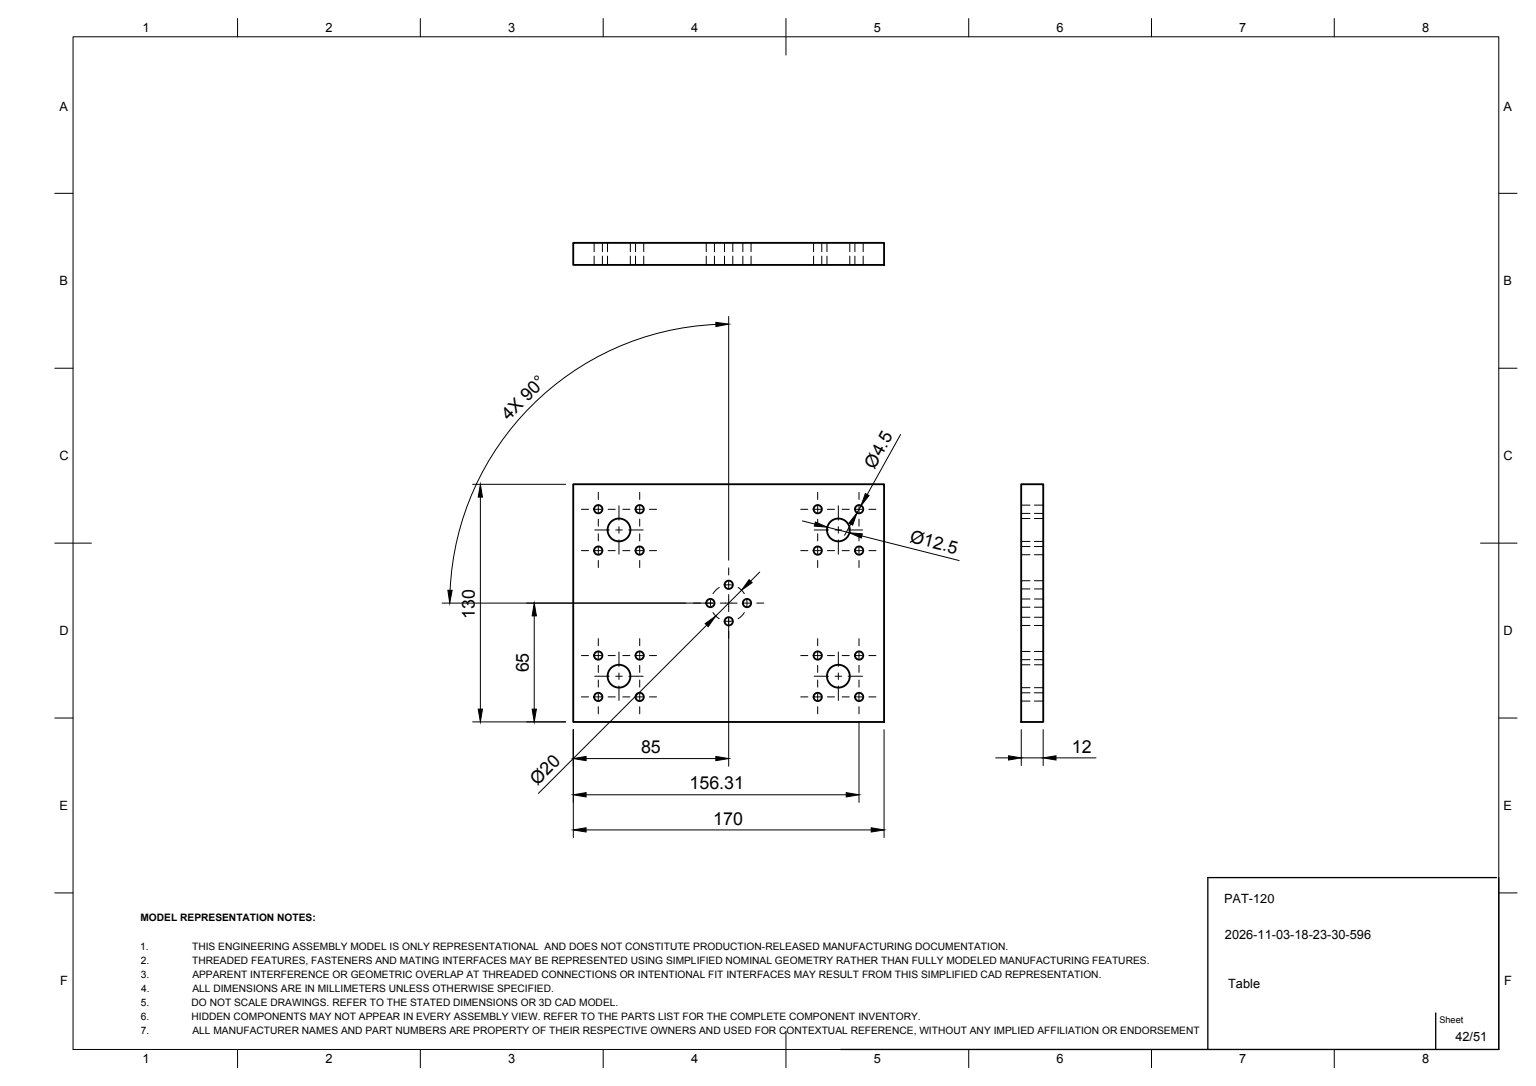
ISO-10303-21;
HEADER;
/* Generated by software containing ST-Developer
 * from STEP Tools, Inc. (www.steptools.com) 
 */

FILE_DESCRIPTION(
/* description */ ('Vibration shaker table dummy'),
/* implementation_level */ '2;1');

FILE_NAME(
/* name */ 'Table.step',
/* time_stamp */ '2026-10-27T10:55:14-07:00',
/* author */ (''),
/* organization */ (''),
/* preprocessor_version */ 'ST-DEVELOPER v20.2',
/* originating_system */ 'Autodesk Translation Framework v15.17.0.0',
/* authorisation */ '');

FILE_SCHEMA (('AUTOMOTIVE_DESIGN { 1 0 10303 214 3 1 1 }'));
ENDSEC;

DATA;
#10=MECHANICAL_DESIGN_GEOMETRIC_PRESENTATION_REPRESENTATION('',(#723),#22394);
#631=SHAPE_REPRESENTATION_RELATIONSHIP('SRR','None',#22678,#677);
#677=ADVANCED_BREP_SHAPE_REPRESENTATION('',(#767),#22384);
#723=STYLED_ITEM('',(#22975),#767);
#767=MANIFOLD_SOLID_BREP('Body1',#9243);
#959=FACE_BOUND('',#2405,.T.);
#960=FACE_BOUND('',#2406,.T.);
#961=FACE_BOUND('',#2407,.T.);
#962=FACE_BOUND('',#2408,.T.);
#963=FACE_BOUND('',#2409,.T.);
#964=FACE_BOUND('',#2410,.T.);
#965=FACE_BOUND('',#2411,.T.);
#966=FACE_BOUND('',#2412,.T.);
#967=FACE_BOUND('',#2413,.T.);
#968=FACE_BOUND('',#2414,.T.);
#969=FACE_BOUND('',#2415,.T.);
#970=FACE_BOUND('',#2416,.T.);
#971=FACE_BOUND('',#2417,.T.);
#972=FACE_BOUND('',#2418,.T.);
#973=FACE_BOUND('',#2419,.T.);
#974=FACE_BOUND('',#2420,.T.);
#975=FACE_BOUND('',#2421,.T.);
#976=FACE_BOUND('',#2422,.T.);
#977=FACE_BOUND('',#2423,.T.);
#978=FACE_BOUND('',#2424,.T.);
#979=FACE_BOUND('',#2425,.T.);
#980=FACE_BOUND('',#2426,.T.);
#981=FACE_BOUND('',#2427,.T.);
#982=FACE_BOUND('',#2428,.T.);
#983=FACE_BOUND('',#2430,.T.);
#984=FACE_BOUND('',#2431,.T.);
#985=FACE_BOUND('',#2432,.T.);
#986=FACE_BOUND('',#2433,.T.);
#987=FACE_BOUND('',#2434,.T.);
#988=FACE_BOUND('',#2435,.T.);
#989=FACE_BOUND('',#2436,.T.);
#990=FACE_BOUND('',#2437,.T.);
#991=FACE_BOUND('',#2438,.T.);
#992=FACE_BOUND('',#2439,.T.);
#993=FACE_BOUND('',#2440,.T.);
#994=FACE_BOUND('',#2441,.T.);
#995=FACE_BOUND('',#2442,.T.);
#996=FACE_BOUND('',#2443,.T.);
#997=FACE_BOUND('',#2444,.T.);
#998=FACE_BOUND('',#2445,.T.);
#999=FACE_BOUND('',#2446,.T.);
#1000=FACE_BOUND('',#2447,.T.);
#1001=FACE_BOUND('',#2448,.T.);
#1002=FACE_BOUND('',#2449,.T.);
#1003=FACE_BOUND('',#2450,.T.);
#1004=FACE_BOUND('',#2451,.T.);
#1005=FACE_BOUND('',#2452,.T.);
#1006=FACE_BOUND('',#2453,.T.);
#1272=PLANE('',#10511);
#1273=PLANE('',#10512);
#1274=PLANE('',#10513);
#1275=PLANE('',#10514);
#1276=PLANE('',#10515);
#1277=PLANE('',#10516);
#1694=FACE_OUTER_BOUND('',#2376,.T.);
#1695=FACE_OUTER_BOUND('',#2377,.T.);
#1696=FACE_OUTER_BOUND('',#2378,.T.);
#1697=FACE_OUTER_BOUND('',#2379,.T.);
#1698=FACE_OUTER_BOUND('',#2380,.T.);
#1699=FACE_OUTER_BOUND('',#2381,.T.);
#1700=FACE_OUTER_BOUND('',#2382,.T.);
#1701=FACE_OUTER_BOUND('',#2383,.T.);
#1702=FACE_OUTER_BOUND('',#2384,.T.);
#1703=FACE_OUTER_BOUND('',#2385,.T.);
#1704=FACE_OUTER_BOUND('',#2386,.T.);
#1705=FACE_OUTER_BOUND('',#2387,.T.);
#1706=FACE_OUTER_BOUND('',#2388,.T.);
#1707=FACE_OUTER_BOUND('',#2389,.T.);
#1708=FACE_OUTER_BOUND('',#2390,.T.);
#1709=FACE_OUTER_BOUND('',#2391,.T.);
#1710=FACE_OUTER_BOUND('',#2392,.T.);
#1711=FACE_OUTER_BOUND('',#2393,.T.);
#1712=FACE_OUTER_BOUND('',#2394,.T.);
#1713=FACE_OUTER_BOUND('',#2395,.T.);
#1714=FACE_OUTER_BOUND('',#2396,.T.);
#1715=FACE_OUTER_BOUND('',#2397,.T.);
#1716=FACE_OUTER_BOUND('',#2398,.T.);
#1717=FACE_OUTER_BOUND('',#2399,.T.);
#1718=FACE_OUTER_BOUND('',#2400,.T.);
#1719=FACE_OUTER_BOUND('',#2401,.T.);
#1720=FACE_OUTER_BOUND('',#2402,.T.);
#1721=FACE_OUTER_BOUND('',#2403,.T.);
#1722=FACE_OUTER_BOUND('',#2404,.T.);
#1723=FACE_OUTER_BOUND('',#2429,.T.);
#2376=EDGE_LOOP('',(#7758,#7759,#7760,#7761));
#2377=EDGE_LOOP('',(#7762,#7763,#7764,#7765));
#2378=EDGE_LOOP('',(#7766,#7767,#7768,#7769));
#2379=EDGE_LOOP('',(#7770,#7771,#7772,#7773));
#2380=EDGE_LOOP('',(#7774,#7775,#7776,#7777));
#2381=EDGE_LOOP('',(#7778,#7779,#7780,#7781));
#2382=EDGE_LOOP('',(#7782,#7783,#7784,#7785));
#2383=EDGE_LOOP('',(#7786,#7787,#7788,#7789));
#2384=EDGE_LOOP('',(#7790,#7791,#7792,#7793));
#2385=EDGE_LOOP('',(#7794,#7795,#7796,#7797));
#2386=EDGE_LOOP('',(#7798,#7799,#7800,#7801));
#2387=EDGE_LOOP('',(#7802,#7803,#7804,#7805));
#2388=EDGE_LOOP('',(#7806,#7807,#7808,#7809));
#2389=EDGE_LOOP('',(#7810,#7811,#7812,#7813));
#2390=EDGE_LOOP('',(#7814,#7815,#7816,#7817));
#2391=EDGE_LOOP('',(#7818,#7819,#7820,#7821));
#2392=EDGE_LOOP('',(#7822,#7823,#7824,#7825));
#2393=EDGE_LOOP('',(#7826,#7827,#7828,#7829));
#2394=EDGE_LOOP('',(#7830,#7831,#7832,#7833));
#2395=EDGE_LOOP('',(#7834,#7835,#7836,#7837));
#2396=EDGE_LOOP('',(#7838,#7839,#7840,#7841));
#2397=EDGE_LOOP('',(#7842,#7843,#7844,#7845));
#2398=EDGE_LOOP('',(#7846,#7847,#7848,#7849));
#2399=EDGE_LOOP('',(#7850,#7851,#7852,#7853));
#2400=EDGE_LOOP('',(#7854,#7855,#7856,#7857));
#2401=EDGE_LOOP('',(#7858,#7859,#7860,#7861));
#2402=EDGE_LOOP('',(#7862,#7863,#7864,#7865));
#2403=EDGE_LOOP('',(#7866,#7867,#7868,#7869));
#2404=EDGE_LOOP('',(#7870,#7871,#7872,#7873));
#2405=EDGE_LOOP('',(#7874));
#2406=EDGE_LOOP('',(#7875));
#2407=EDGE_LOOP('',(#7876));
#2408=EDGE_LOOP('',(#7877));
#2409=EDGE_LOOP('',(#7878));
#2410=EDGE_LOOP('',(#7879));
#2411=EDGE_LOOP('',(#7880));
#2412=EDGE_LOOP('',(#7881));
#2413=EDGE_LOOP('',(#7882));
#2414=EDGE_LOOP('',(#7883));
#2415=EDGE_LOOP('',(#7884));
#2416=EDGE_LOOP('',(#7885));
#2417=EDGE_LOOP('',(#7886));
#2418=EDGE_LOOP('',(#7887));
#2419=EDGE_LOOP('',(#7888));
#2420=EDGE_LOOP('',(#7889));
#2421=EDGE_LOOP('',(#7890));
#2422=EDGE_LOOP('',(#7891));
#2423=EDGE_LOOP('',(#7892));
#2424=EDGE_LOOP('',(#7893));
#2425=EDGE_LOOP('',(#7894));
#2426=EDGE_LOOP('',(#7895));
#2427=EDGE_LOOP('',(#7896));
#2428=EDGE_LOOP('',(#7897));
#2429=EDGE_LOOP('',(#7898,#7899,#7900,#7901));
#2430=EDGE_LOOP('',(#7902));
#2431=EDGE_LOOP('',(#7903));
#2432=EDGE_LOOP('',(#7904));
#2433=EDGE_LOOP('',(#7905));
#2434=EDGE_LOOP('',(#7906));
#2435=EDGE_LOOP('',(#7907));
#2436=EDGE_LOOP('',(#7908));
#2437=EDGE_LOOP('',(#7909));
#2438=EDGE_LOOP('',(#7910));
#2439=EDGE_LOOP('',(#7911));
#2440=EDGE_LOOP('',(#7912));
#2441=EDGE_LOOP('',(#7913));
#2442=EDGE_LOOP('',(#7914));
#2443=EDGE_LOOP('',(#7915));
#2444=EDGE_LOOP('',(#7916));
#2445=EDGE_LOOP('',(#7917));
#2446=EDGE_LOOP('',(#7918));
#2447=EDGE_LOOP('',(#7919));
#2448=EDGE_LOOP('',(#7920));
#2449=EDGE_LOOP('',(#7921));
#2450=EDGE_LOOP('',(#7922));
#2451=EDGE_LOOP('',(#7923));
#2452=EDGE_LOOP('',(#7924));
#2453=EDGE_LOOP('',(#7925));
#3085=LINE('',#21382,#3704);
#3086=LINE('',#21388,#3705);
#3087=LINE('',#21394,#3706);
#3088=LINE('',#21400,#3707);
#3089=LINE('',#21406,#3708);
#3090=LINE('',#21412,#3709);
#3091=LINE('',#21418,#3710);
#3092=LINE('',#21424,#3711);
#3093=LINE('',#21430,#3712);
#3094=LINE('',#21436,#3713);
#3095=LINE('',#21442,#3714);
#3096=LINE('',#21448,#3715);
#3097=LINE('',#21454,#3716);
#3098=LINE('',#21460,#3717);
#3099=LINE('',#21466,#3718);
#3100=LINE('',#21472,#3719);
#3101=LINE('',#21478,#3720);
#3102=LINE('',#21484,#3721);
#3103=LINE('',#21490,#3722);
#3104=LINE('',#21496,#3723);
#3105=LINE('',#21502,#3724);
#3106=LINE('',#21508,#3725);
#3107=LINE('',#21514,#3726);
#3108=LINE('',#21520,#3727);
#3109=LINE('',#21525,#3728);
#3110=LINE('',#21527,#3729);
#3111=LINE('',#21529,#3730);
#3112=LINE('',#21530,#3731);
#3113=LINE('',#21533,#3732);
#3114=LINE('',#21535,#3733);
#3115=LINE('',#21536,#3734);
#3116=LINE('',#21539,#3735);
#3117=LINE('',#21541,#3736);
#3118=LINE('',#21542,#3737);
#3119=LINE('',#21544,#3738);
#3120=LINE('',#21545,#3739);
#3704=VECTOR('',#12775,0.225);
#3705=VECTOR('',#12782,0.225);
#3706=VECTOR('',#12789,0.225);
#3707=VECTOR('',#12796,0.225);
#3708=VECTOR('',#12803,0.225);
#3709=VECTOR('',#12810,0.225);
#3710=VECTOR('',#12817,0.225);
#3711=VECTOR('',#12824,0.225);
#3712=VECTOR('',#12831,0.225);
#3713=VECTOR('',#12838,0.225);
#3714=VECTOR('',#12845,0.225);
#3715=VECTOR('',#12852,0.225);
#3716=VECTOR('',#12859,0.225);
#3717=VECTOR('',#12866,0.225);
#3718=VECTOR('',#12873,0.225);
#3719=VECTOR('',#12880,0.225);
#3720=VECTOR('',#12887,0.225);
#3721=VECTOR('',#12894,0.225);
#3722=VECTOR('',#12901,0.225);
#3723=VECTOR('',#12908,0.225);
#3724=VECTOR('',#12915,0.625);
#3725=VECTOR('',#12922,0.625);
#3726=VECTOR('',#12929,0.625);
#3727=VECTOR('',#12936,0.625);
#3728=VECTOR('',#12941,1.);
#3729=VECTOR('',#12942,1.);
#3730=VECTOR('',#12943,1.);
#3731=VECTOR('',#12944,1.);
#3732=VECTOR('',#12947,1.);
#3733=VECTOR('',#12948,1.);
#3734=VECTOR('',#12949,1.);
#3735=VECTOR('',#12952,1.);
#3736=VECTOR('',#12953,1.);
#3737=VECTOR('',#12954,1.);
#3738=VECTOR('',#12957,1.);
#3739=VECTOR('',#12958,1.);
#4149=CIRCLE('',#10440,0.225);
#4150=CIRCLE('',#10441,0.225);
#4151=CIRCLE('',#10443,0.225);
#4152=CIRCLE('',#10444,0.225);
#4153=CIRCLE('',#10446,0.225);
#4154=CIRCLE('',#10447,0.225);
#4155=CIRCLE('',#10449,0.225);
#4156=CIRCLE('',#10450,0.225);
#4157=CIRCLE('',#10452,0.225);
#4158=CIRCLE('',#10453,0.225);
#4159=CIRCLE('',#10455,0.225);
#4160=CIRCLE('',#10456,0.225);
#4161=CIRCLE('',#10458,0.225);
#4162=CIRCLE('',#10459,0.225);
#4163=CIRCLE('',#10461,0.225);
#4164=CIRCLE('',#10462,0.225);
#4165=CIRCLE('',#10464,0.225);
#4166=CIRCLE('',#10465,0.225);
#4167=CIRCLE('',#10467,0.225);
#4168=CIRCLE('',#10468,0.225);
#4169=CIRCLE('',#10470,0.225);
#4170=CIRCLE('',#10471,0.225);
#4171=CIRCLE('',#10473,0.225);
#4172=CIRCLE('',#10474,0.225);
#4173=CIRCLE('',#10476,0.225);
#4174=CIRCLE('',#10477,0.225);
#4175=CIRCLE('',#10479,0.225);
#4176=CIRCLE('',#10480,0.225);
#4177=CIRCLE('',#10482,0.225);
#4178=CIRCLE('',#10483,0.225);
#4179=CIRCLE('',#10485,0.225);
#4180=CIRCLE('',#10486,0.225);
#4181=CIRCLE('',#10488,0.225);
#4182=CIRCLE('',#10489,0.225);
#4183=CIRCLE('',#10491,0.225);
#4184=CIRCLE('',#10492,0.225);
#4185=CIRCLE('',#10494,0.225);
#4186=CIRCLE('',#10495,0.225);
#4187=CIRCLE('',#10497,0.225);
#4188=CIRCLE('',#10498,0.225);
#4189=CIRCLE('',#10500,0.625);
#4190=CIRCLE('',#10501,0.625);
#4191=CIRCLE('',#10503,0.625);
#4192=CIRCLE('',#10504,0.625);
#4193=CIRCLE('',#10506,0.625);
#4194=CIRCLE('',#10507,0.625);
#4195=CIRCLE('',#10509,0.625);
#4196=CIRCLE('',#10510,0.625);
#4868=VERTEX_POINT('',#21379);
#4869=VERTEX_POINT('',#21381);
#4870=VERTEX_POINT('',#21385);
#4871=VERTEX_POINT('',#21387);
#4872=VERTEX_POINT('',#21391);
#4873=VERTEX_POINT('',#21393);
#4874=VERTEX_POINT('',#21397);
#4875=VERTEX_POINT('',#21399);
#4876=VERTEX_POINT('',#21403);
#4877=VERTEX_POINT('',#21405);
#4878=VERTEX_POINT('',#21409);
#4879=VERTEX_POINT('',#21411);
#4880=VERTEX_POINT('',#21415);
#4881=VERTEX_POINT('',#21417);
#4882=VERTEX_POINT('',#21421);
#4883=VERTEX_POINT('',#21423);
#4884=VERTEX_POINT('',#21427);
#4885=VERTEX_POINT('',#21429);
#4886=VERTEX_POINT('',#21433);
#4887=VERTEX_POINT('',#21435);
#4888=VERTEX_POINT('',#21439);
#4889=VERTEX_POINT('',#21441);
#4890=VERTEX_POINT('',#21445);
#4891=VERTEX_POINT('',#21447);
#4892=VERTEX_POINT('',#21451);
#4893=VERTEX_POINT('',#21453);
#4894=VERTEX_POINT('',#21457);
#4895=VERTEX_POINT('',#21459);
#4896=VERTEX_POINT('',#21463);
#4897=VERTEX_POINT('',#21465);
#4898=VERTEX_POINT('',#21469);
#4899=VERTEX_POINT('',#21471);
#4900=VERTEX_POINT('',#21475);
#4901=VERTEX_POINT('',#21477);
#4902=VERTEX_POINT('',#21481);
#4903=VERTEX_POINT('',#21483);
#4904=VERTEX_POINT('',#21487);
#4905=VERTEX_POINT('',#21489);
#4906=VERTEX_POINT('',#21493);
#4907=VERTEX_POINT('',#21495);
#4908=VERTEX_POINT('',#21499);
#4909=VERTEX_POINT('',#21501);
#4910=VERTEX_POINT('',#21505);
#4911=VERTEX_POINT('',#21507);
#4912=VERTEX_POINT('',#21511);
#4913=VERTEX_POINT('',#21513);
#4914=VERTEX_POINT('',#21517);
#4915=VERTEX_POINT('',#21519);
#4916=VERTEX_POINT('',#21523);
#4917=VERTEX_POINT('',#21524);
#4918=VERTEX_POINT('',#21526);
#4919=VERTEX_POINT('',#21528);
#4920=VERTEX_POINT('',#21532);
#4921=VERTEX_POINT('',#21534);
#4922=VERTEX_POINT('',#21538);
#4923=VERTEX_POINT('',#21540);
#5872=EDGE_CURVE('',#4868,#4868,#4149,.T.);
#5873=EDGE_CURVE('',#4868,#4869,#3085,.T.);
#5874=EDGE_CURVE('',#4869,#4869,#4150,.T.);
#5875=EDGE_CURVE('',#4870,#4870,#4151,.T.);
#5876=EDGE_CURVE('',#4870,#4871,#3086,.T.);
#5877=EDGE_CURVE('',#4871,#4871,#4152,.T.);
#5878=EDGE_CURVE('',#4872,#4872,#4153,.T.);
#5879=EDGE_CURVE('',#4872,#4873,#3087,.T.);
#5880=EDGE_CURVE('',#4873,#4873,#4154,.T.);
#5881=EDGE_CURVE('',#4874,#4874,#4155,.T.);
#5882=EDGE_CURVE('',#4874,#4875,#3088,.T.);
#5883=EDGE_CURVE('',#4875,#4875,#4156,.T.);
#5884=EDGE_CURVE('',#4876,#4876,#4157,.T.);
#5885=EDGE_CURVE('',#4876,#4877,#3089,.T.);
#5886=EDGE_CURVE('',#4877,#4877,#4158,.T.);
#5887=EDGE_CURVE('',#4878,#4878,#4159,.T.);
#5888=EDGE_CURVE('',#4878,#4879,#3090,.T.);
#5889=EDGE_CURVE('',#4879,#4879,#4160,.T.);
#5890=EDGE_CURVE('',#4880,#4880,#4161,.T.);
#5891=EDGE_CURVE('',#4880,#4881,#3091,.T.);
#5892=EDGE_CURVE('',#4881,#4881,#4162,.T.);
#5893=EDGE_CURVE('',#4882,#4882,#4163,.T.);
#5894=EDGE_CURVE('',#4882,#4883,#3092,.T.);
#5895=EDGE_CURVE('',#4883,#4883,#4164,.T.);
#5896=EDGE_CURVE('',#4884,#4884,#4165,.T.);
#5897=EDGE_CURVE('',#4884,#4885,#3093,.T.);
#5898=EDGE_CURVE('',#4885,#4885,#4166,.T.);
#5899=EDGE_CURVE('',#4886,#4886,#4167,.T.);
#5900=EDGE_CURVE('',#4886,#4887,#3094,.T.);
#5901=EDGE_CURVE('',#4887,#4887,#4168,.T.);
#5902=EDGE_CURVE('',#4888,#4888,#4169,.T.);
#5903=EDGE_CURVE('',#4888,#4889,#3095,.T.);
#5904=EDGE_CURVE('',#4889,#4889,#4170,.T.);
#5905=EDGE_CURVE('',#4890,#4890,#4171,.T.);
#5906=EDGE_CURVE('',#4890,#4891,#3096,.T.);
#5907=EDGE_CURVE('',#4891,#4891,#4172,.T.);
#5908=EDGE_CURVE('',#4892,#4892,#4173,.T.);
#5909=EDGE_CURVE('',#4892,#4893,#3097,.T.);
#5910=EDGE_CURVE('',#4893,#4893,#4174,.T.);
#5911=EDGE_CURVE('',#4894,#4894,#4175,.T.);
#5912=EDGE_CURVE('',#4894,#4895,#3098,.T.);
#5913=EDGE_CURVE('',#4895,#4895,#4176,.T.);
#5914=EDGE_CURVE('',#4896,#4896,#4177,.T.);
#5915=EDGE_CURVE('',#4896,#4897,#3099,.T.);
#5916=EDGE_CURVE('',#4897,#4897,#4178,.T.);
#5917=EDGE_CURVE('',#4898,#4898,#4179,.T.);
#5918=EDGE_CURVE('',#4898,#4899,#3100,.T.);
#5919=EDGE_CURVE('',#4899,#4899,#4180,.T.);
#5920=EDGE_CURVE('',#4900,#4900,#4181,.T.);
#5921=EDGE_CURVE('',#4900,#4901,#3101,.T.);
#5922=EDGE_CURVE('',#4901,#4901,#4182,.T.);
#5923=EDGE_CURVE('',#4902,#4902,#4183,.T.);
#5924=EDGE_CURVE('',#4902,#4903,#3102,.T.);
#5925=EDGE_CURVE('',#4903,#4903,#4184,.T.);
#5926=EDGE_CURVE('',#4904,#4904,#4185,.T.);
#5927=EDGE_CURVE('',#4904,#4905,#3103,.T.);
#5928=EDGE_CURVE('',#4905,#4905,#4186,.T.);
#5929=EDGE_CURVE('',#4906,#4906,#4187,.T.);
#5930=EDGE_CURVE('',#4906,#4907,#3104,.T.);
#5931=EDGE_CURVE('',#4907,#4907,#4188,.T.);
#5932=EDGE_CURVE('',#4908,#4908,#4189,.T.);
#5933=EDGE_CURVE('',#4908,#4909,#3105,.T.);
#5934=EDGE_CURVE('',#4909,#4909,#4190,.T.);
#5935=EDGE_CURVE('',#4910,#4910,#4191,.T.);
#5936=EDGE_CURVE('',#4910,#4911,#3106,.T.);
#5937=EDGE_CURVE('',#4911,#4911,#4192,.T.);
#5938=EDGE_CURVE('',#4912,#4912,#4193,.T.);
#5939=EDGE_CURVE('',#4912,#4913,#3107,.T.);
#5940=EDGE_CURVE('',#4913,#4913,#4194,.T.);
#5941=EDGE_CURVE('',#4914,#4914,#4195,.T.);
#5942=EDGE_CURVE('',#4914,#4915,#3108,.T.);
#5943=EDGE_CURVE('',#4915,#4915,#4196,.T.);
#5944=EDGE_CURVE('',#4916,#4917,#3109,.T.);
#5945=EDGE_CURVE('',#4917,#4918,#3110,.T.);
#5946=EDGE_CURVE('',#4919,#4918,#3111,.T.);
#5947=EDGE_CURVE('',#4916,#4919,#3112,.T.);
#5948=EDGE_CURVE('',#4920,#4916,#3113,.T.);
#5949=EDGE_CURVE('',#4921,#4919,#3114,.T.);
#5950=EDGE_CURVE('',#4920,#4921,#3115,.T.);
#5951=EDGE_CURVE('',#4922,#4920,#3116,.T.);
#5952=EDGE_CURVE('',#4923,#4921,#3117,.T.);
#5953=EDGE_CURVE('',#4922,#4923,#3118,.T.);
#5954=EDGE_CURVE('',#4917,#4922,#3119,.T.);
#5955=EDGE_CURVE('',#4918,#4923,#3120,.T.);
#7758=ORIENTED_EDGE('',*,*,#5872,.F.);
#7759=ORIENTED_EDGE('',*,*,#5873,.T.);
#7760=ORIENTED_EDGE('',*,*,#5874,.F.);
#7761=ORIENTED_EDGE('',*,*,#5873,.F.);
#7762=ORIENTED_EDGE('',*,*,#5875,.F.);
#7763=ORIENTED_EDGE('',*,*,#5876,.T.);
#7764=ORIENTED_EDGE('',*,*,#5877,.F.);
#7765=ORIENTED_EDGE('',*,*,#5876,.F.);
#7766=ORIENTED_EDGE('',*,*,#5878,.F.);
#7767=ORIENTED_EDGE('',*,*,#5879,.T.);
#7768=ORIENTED_EDGE('',*,*,#5880,.F.);
#7769=ORIENTED_EDGE('',*,*,#5879,.F.);
#7770=ORIENTED_EDGE('',*,*,#5881,.F.);
#7771=ORIENTED_EDGE('',*,*,#5882,.T.);
#7772=ORIENTED_EDGE('',*,*,#5883,.F.);
#7773=ORIENTED_EDGE('',*,*,#5882,.F.);
#7774=ORIENTED_EDGE('',*,*,#5884,.F.);
#7775=ORIENTED_EDGE('',*,*,#5885,.T.);
#7776=ORIENTED_EDGE('',*,*,#5886,.F.);
#7777=ORIENTED_EDGE('',*,*,#5885,.F.);
#7778=ORIENTED_EDGE('',*,*,#5887,.F.);
#7779=ORIENTED_EDGE('',*,*,#5888,.T.);
#7780=ORIENTED_EDGE('',*,*,#5889,.F.);
#7781=ORIENTED_EDGE('',*,*,#5888,.F.);
#7782=ORIENTED_EDGE('',*,*,#5890,.F.);
#7783=ORIENTED_EDGE('',*,*,#5891,.T.);
#7784=ORIENTED_EDGE('',*,*,#5892,.F.);
#7785=ORIENTED_EDGE('',*,*,#5891,.F.);
#7786=ORIENTED_EDGE('',*,*,#5893,.F.);
#7787=ORIENTED_EDGE('',*,*,#5894,.T.);
#7788=ORIENTED_EDGE('',*,*,#5895,.F.);
#7789=ORIENTED_EDGE('',*,*,#5894,.F.);
#7790=ORIENTED_EDGE('',*,*,#5896,.F.);
#7791=ORIENTED_EDGE('',*,*,#5897,.T.);
#7792=ORIENTED_EDGE('',*,*,#5898,.F.);
#7793=ORIENTED_EDGE('',*,*,#5897,.F.);
#7794=ORIENTED_EDGE('',*,*,#5899,.F.);
#7795=ORIENTED_EDGE('',*,*,#5900,.T.);
#7796=ORIENTED_EDGE('',*,*,#5901,.F.);
#7797=ORIENTED_EDGE('',*,*,#5900,.F.);
#7798=ORIENTED_EDGE('',*,*,#5902,.F.);
#7799=ORIENTED_EDGE('',*,*,#5903,.T.);
#7800=ORIENTED_EDGE('',*,*,#5904,.F.);
#7801=ORIENTED_EDGE('',*,*,#5903,.F.);
#7802=ORIENTED_EDGE('',*,*,#5905,.F.);
#7803=ORIENTED_EDGE('',*,*,#5906,.T.);
#7804=ORIENTED_EDGE('',*,*,#5907,.F.);
#7805=ORIENTED_EDGE('',*,*,#5906,.F.);
#7806=ORIENTED_EDGE('',*,*,#5908,.F.);
#7807=ORIENTED_EDGE('',*,*,#5909,.T.);
#7808=ORIENTED_EDGE('',*,*,#5910,.F.);
#7809=ORIENTED_EDGE('',*,*,#5909,.F.);
#7810=ORIENTED_EDGE('',*,*,#5911,.F.);
#7811=ORIENTED_EDGE('',*,*,#5912,.T.);
#7812=ORIENTED_EDGE('',*,*,#5913,.F.);
#7813=ORIENTED_EDGE('',*,*,#5912,.F.);
#7814=ORIENTED_EDGE('',*,*,#5914,.F.);
#7815=ORIENTED_EDGE('',*,*,#5915,.T.);
#7816=ORIENTED_EDGE('',*,*,#5916,.F.);
#7817=ORIENTED_EDGE('',*,*,#5915,.F.);
#7818=ORIENTED_EDGE('',*,*,#5917,.F.);
#7819=ORIENTED_EDGE('',*,*,#5918,.T.);
#7820=ORIENTED_EDGE('',*,*,#5919,.F.);
#7821=ORIENTED_EDGE('',*,*,#5918,.F.);
#7822=ORIENTED_EDGE('',*,*,#5920,.F.);
#7823=ORIENTED_EDGE('',*,*,#5921,.T.);
#7824=ORIENTED_EDGE('',*,*,#5922,.F.);
#7825=ORIENTED_EDGE('',*,*,#5921,.F.);
#7826=ORIENTED_EDGE('',*,*,#5923,.F.);
#7827=ORIENTED_EDGE('',*,*,#5924,.T.);
#7828=ORIENTED_EDGE('',*,*,#5925,.F.);
#7829=ORIENTED_EDGE('',*,*,#5924,.F.);
#7830=ORIENTED_EDGE('',*,*,#5926,.F.);
#7831=ORIENTED_EDGE('',*,*,#5927,.T.);
#7832=ORIENTED_EDGE('',*,*,#5928,.F.);
#7833=ORIENTED_EDGE('',*,*,#5927,.F.);
#7834=ORIENTED_EDGE('',*,*,#5929,.F.);
#7835=ORIENTED_EDGE('',*,*,#5930,.T.);
#7836=ORIENTED_EDGE('',*,*,#5931,.F.);
#7837=ORIENTED_EDGE('',*,*,#5930,.F.);
#7838=ORIENTED_EDGE('',*,*,#5932,.F.);
#7839=ORIENTED_EDGE('',*,*,#5933,.T.);
#7840=ORIENTED_EDGE('',*,*,#5934,.F.);
#7841=ORIENTED_EDGE('',*,*,#5933,.F.);
#7842=ORIENTED_EDGE('',*,*,#5935,.F.);
#7843=ORIENTED_EDGE('',*,*,#5936,.T.);
#7844=ORIENTED_EDGE('',*,*,#5937,.F.);
#7845=ORIENTED_EDGE('',*,*,#5936,.F.);
#7846=ORIENTED_EDGE('',*,*,#5938,.F.);
#7847=ORIENTED_EDGE('',*,*,#5939,.T.);
#7848=ORIENTED_EDGE('',*,*,#5940,.F.);
#7849=ORIENTED_EDGE('',*,*,#5939,.F.);
#7850=ORIENTED_EDGE('',*,*,#5941,.F.);
#7851=ORIENTED_EDGE('',*,*,#5942,.T.);
#7852=ORIENTED_EDGE('',*,*,#5943,.F.);
#7853=ORIENTED_EDGE('',*,*,#5942,.F.);
#7854=ORIENTED_EDGE('',*,*,#5944,.T.);
#7855=ORIENTED_EDGE('',*,*,#5945,.T.);
#7856=ORIENTED_EDGE('',*,*,#5946,.F.);
#7857=ORIENTED_EDGE('',*,*,#5947,.F.);
#7858=ORIENTED_EDGE('',*,*,#5948,.T.);
#7859=ORIENTED_EDGE('',*,*,#5947,.T.);
#7860=ORIENTED_EDGE('',*,*,#5949,.F.);
#7861=ORIENTED_EDGE('',*,*,#5950,.F.);
#7862=ORIENTED_EDGE('',*,*,#5951,.T.);
#7863=ORIENTED_EDGE('',*,*,#5950,.T.);
#7864=ORIENTED_EDGE('',*,*,#5952,.F.);
#7865=ORIENTED_EDGE('',*,*,#5953,.F.);
#7866=ORIENTED_EDGE('',*,*,#5954,.T.);
#7867=ORIENTED_EDGE('',*,*,#5953,.T.);
#7868=ORIENTED_EDGE('',*,*,#5955,.F.);
#7869=ORIENTED_EDGE('',*,*,#5945,.F.);
#7870=ORIENTED_EDGE('',*,*,#5955,.T.);
#7871=ORIENTED_EDGE('',*,*,#5952,.T.);
#7872=ORIENTED_EDGE('',*,*,#5949,.T.);
#7873=ORIENTED_EDGE('',*,*,#5946,.T.);
#7874=ORIENTED_EDGE('',*,*,#5886,.T.);
#7875=ORIENTED_EDGE('',*,*,#5889,.T.);
#7876=ORIENTED_EDGE('',*,*,#5892,.T.);
#7877=ORIENTED_EDGE('',*,*,#5895,.T.);
#7878=ORIENTED_EDGE('',*,*,#5910,.T.);
#7879=ORIENTED_EDGE('',*,*,#5913,.T.);
#7880=ORIENTED_EDGE('',*,*,#5916,.T.);
#7881=ORIENTED_EDGE('',*,*,#5919,.T.);
#7882=ORIENTED_EDGE('',*,*,#5943,.T.);
#7883=ORIENTED_EDGE('',*,*,#5940,.T.);
#7884=ORIENTED_EDGE('',*,*,#5937,.T.);
#7885=ORIENTED_EDGE('',*,*,#5934,.T.);
#7886=ORIENTED_EDGE('',*,*,#5931,.T.);
#7887=ORIENTED_EDGE('',*,*,#5928,.T.);
#7888=ORIENTED_EDGE('',*,*,#5925,.T.);
#7889=ORIENTED_EDGE('',*,*,#5922,.T.);
#7890=ORIENTED_EDGE('',*,*,#5907,.T.);
#7891=ORIENTED_EDGE('',*,*,#5904,.T.);
#7892=ORIENTED_EDGE('',*,*,#5901,.T.);
#7893=ORIENTED_EDGE('',*,*,#5898,.T.);
#7894=ORIENTED_EDGE('',*,*,#5883,.T.);
#7895=ORIENTED_EDGE('',*,*,#5880,.T.);
#7896=ORIENTED_EDGE('',*,*,#5877,.T.);
#7897=ORIENTED_EDGE('',*,*,#5874,.T.);
#7898=ORIENTED_EDGE('',*,*,#5954,.F.);
#7899=ORIENTED_EDGE('',*,*,#5944,.F.);
#7900=ORIENTED_EDGE('',*,*,#5948,.F.);
#7901=ORIENTED_EDGE('',*,*,#5951,.F.);
#7902=ORIENTED_EDGE('',*,*,#5884,.T.);
#7903=ORIENTED_EDGE('',*,*,#5887,.T.);
#7904=ORIENTED_EDGE('',*,*,#5890,.T.);
#7905=ORIENTED_EDGE('',*,*,#5893,.T.);
#7906=ORIENTED_EDGE('',*,*,#5908,.T.);
#7907=ORIENTED_EDGE('',*,*,#5911,.T.);
#7908=ORIENTED_EDGE('',*,*,#5914,.T.);
#7909=ORIENTED_EDGE('',*,*,#5917,.T.);
#7910=ORIENTED_EDGE('',*,*,#5941,.T.);
#7911=ORIENTED_EDGE('',*,*,#5938,.T.);
#7912=ORIENTED_EDGE('',*,*,#5935,.T.);
#7913=ORIENTED_EDGE('',*,*,#5932,.T.);
#7914=ORIENTED_EDGE('',*,*,#5929,.T.);
#7915=ORIENTED_EDGE('',*,*,#5926,.T.);
#7916=ORIENTED_EDGE('',*,*,#5923,.T.);
#7917=ORIENTED_EDGE('',*,*,#5920,.T.);
#7918=ORIENTED_EDGE('',*,*,#5905,.T.);
#7919=ORIENTED_EDGE('',*,*,#5902,.T.);
#7920=ORIENTED_EDGE('',*,*,#5899,.T.);
#7921=ORIENTED_EDGE('',*,*,#5896,.T.);
#7922=ORIENTED_EDGE('',*,*,#5881,.T.);
#7923=ORIENTED_EDGE('',*,*,#5878,.T.);
#7924=ORIENTED_EDGE('',*,*,#5875,.T.);
#7925=ORIENTED_EDGE('',*,*,#5872,.T.);
#8634=CYLINDRICAL_SURFACE('',#10439,0.225);
#8635=CYLINDRICAL_SURFACE('',#10442,0.225);
#8636=CYLINDRICAL_SURFACE('',#10445,0.225);
#8637=CYLINDRICAL_SURFACE('',#10448,0.225);
#8638=CYLINDRICAL_SURFACE('',#10451,0.225);
#8639=CYLINDRICAL_SURFACE('',#10454,0.225);
#8640=CYLINDRICAL_SURFACE('',#10457,0.225);
#8641=CYLINDRICAL_SURFACE('',#10460,0.225);
#8642=CYLINDRICAL_SURFACE('',#10463,0.225);
#8643=CYLINDRICAL_SURFACE('',#10466,0.225);
#8644=CYLINDRICAL_SURFACE('',#10469,0.225);
#8645=CYLINDRICAL_SURFACE('',#10472,0.225);
#8646=CYLINDRICAL_SURFACE('',#10475,0.225);
#8647=CYLINDRICAL_SURFACE('',#10478,0.225);
#8648=CYLINDRICAL_SURFACE('',#10481,0.225);
#8649=CYLINDRICAL_SURFACE('',#10484,0.225);
#8650=CYLINDRICAL_SURFACE('',#10487,0.225);
#8651=CYLINDRICAL_SURFACE('',#10490,0.225);
#8652=CYLINDRICAL_SURFACE('',#10493,0.225);
#8653=CYLINDRICAL_SURFACE('',#10496,0.225);
#8654=CYLINDRICAL_SURFACE('',#10499,0.625);
#8655=CYLINDRICAL_SURFACE('',#10502,0.625);
#8656=CYLINDRICAL_SURFACE('',#10505,0.625);
#8657=CYLINDRICAL_SURFACE('',#10508,0.625);
#9059=ADVANCED_FACE('',(#1694),#8634,.F.);
#9060=ADVANCED_FACE('',(#1695),#8635,.F.);
#9061=ADVANCED_FACE('',(#1696),#8636,.F.);
#9062=ADVANCED_FACE('',(#1697),#8637,.F.);
#9063=ADVANCED_FACE('',(#1698),#8638,.F.);
#9064=ADVANCED_FACE('',(#1699),#8639,.F.);
#9065=ADVANCED_FACE('',(#1700),#8640,.F.);
#9066=ADVANCED_FACE('',(#1701),#8641,.F.);
#9067=ADVANCED_FACE('',(#1702),#8642,.F.);
#9068=ADVANCED_FACE('',(#1703),#8643,.F.);
#9069=ADVANCED_FACE('',(#1704),#8644,.F.);
#9070=ADVANCED_FACE('',(#1705),#8645,.F.);
#9071=ADVANCED_FACE('',(#1706),#8646,.F.);
#9072=ADVANCED_FACE('',(#1707),#8647,.F.);
#9073=ADVANCED_FACE('',(#1708),#8648,.F.);
#9074=ADVANCED_FACE('',(#1709),#8649,.F.);
#9075=ADVANCED_FACE('',(#1710),#8650,.F.);
#9076=ADVANCED_FACE('',(#1711),#8651,.F.);
#9077=ADVANCED_FACE('',(#1712),#8652,.F.);
#9078=ADVANCED_FACE('',(#1713),#8653,.F.);
#9079=ADVANCED_FACE('',(#1714),#8654,.F.);
#9080=ADVANCED_FACE('',(#1715),#8655,.F.);
#9081=ADVANCED_FACE('',(#1716),#8656,.F.);
#9082=ADVANCED_FACE('',(#1717),#8657,.F.);
#9083=ADVANCED_FACE('',(#1718),#1272,.T.);
#9084=ADVANCED_FACE('',(#1719),#1273,.T.);
#9085=ADVANCED_FACE('',(#1720),#1274,.T.);
#9086=ADVANCED_FACE('',(#1721),#1275,.T.);
#9087=ADVANCED_FACE('',(#1722,#959,#960,#961,#962,#963,#964,#965,#966,#967,
#968,#969,#970,#971,#972,#973,#974,#975,#976,#977,#978,#979,#980,#981,#982),
#1276,.T.);
#9088=ADVANCED_FACE('',(#1723,#983,#984,#985,#986,#987,#988,#989,#990,#991,
#992,#993,#994,#995,#996,#997,#998,#999,#1000,#1001,#1002,#1003,#1004,#1005,
#1006),#1277,.F.);
#9243=CLOSED_SHELL('',(#9059,#9060,#9061,#9062,#9063,#9064,#9065,#9066,
#9067,#9068,#9069,#9070,#9071,#9072,#9073,#9074,#9075,#9076,#9077,#9078,
#9079,#9080,#9081,#9082,#9083,#9084,#9085,#9086,#9087,#9088));
#10438=AXIS2_PLACEMENT_3D('',#21377,#12769,#12770);
#10439=AXIS2_PLACEMENT_3D('',#21378,#12771,#12772);
#10440=AXIS2_PLACEMENT_3D('',#21380,#12773,#12774);
#10441=AXIS2_PLACEMENT_3D('',#21383,#12776,#12777);
#10442=AXIS2_PLACEMENT_3D('',#21384,#12778,#12779);
#10443=AXIS2_PLACEMENT_3D('',#21386,#12780,#12781);
#10444=AXIS2_PLACEMENT_3D('',#21389,#12783,#12784);
#10445=AXIS2_PLACEMENT_3D('',#21390,#12785,#12786);
#10446=AXIS2_PLACEMENT_3D('',#21392,#12787,#12788);
#10447=AXIS2_PLACEMENT_3D('',#21395,#12790,#12791);
#10448=AXIS2_PLACEMENT_3D('',#21396,#12792,#12793);
#10449=AXIS2_PLACEMENT_3D('',#21398,#12794,#12795);
#10450=AXIS2_PLACEMENT_3D('',#21401,#12797,#12798);
#10451=AXIS2_PLACEMENT_3D('',#21402,#12799,#12800);
#10452=AXIS2_PLACEMENT_3D('',#21404,#12801,#12802);
#10453=AXIS2_PLACEMENT_3D('',#21407,#12804,#12805);
#10454=AXIS2_PLACEMENT_3D('',#21408,#12806,#12807);
#10455=AXIS2_PLACEMENT_3D('',#21410,#12808,#12809);
#10456=AXIS2_PLACEMENT_3D('',#21413,#12811,#12812);
#10457=AXIS2_PLACEMENT_3D('',#21414,#12813,#12814);
#10458=AXIS2_PLACEMENT_3D('',#21416,#12815,#12816);
#10459=AXIS2_PLACEMENT_3D('',#21419,#12818,#12819);
#10460=AXIS2_PLACEMENT_3D('',#21420,#12820,#12821);
#10461=AXIS2_PLACEMENT_3D('',#21422,#12822,#12823);
#10462=AXIS2_PLACEMENT_3D('',#21425,#12825,#12826);
#10463=AXIS2_PLACEMENT_3D('',#21426,#12827,#12828);
#10464=AXIS2_PLACEMENT_3D('',#21428,#12829,#12830);
#10465=AXIS2_PLACEMENT_3D('',#21431,#12832,#12833);
#10466=AXIS2_PLACEMENT_3D('',#21432,#12834,#12835);
#10467=AXIS2_PLACEMENT_3D('',#21434,#12836,#12837);
#10468=AXIS2_PLACEMENT_3D('',#21437,#12839,#12840);
#10469=AXIS2_PLACEMENT_3D('',#21438,#12841,#12842);
#10470=AXIS2_PLACEMENT_3D('',#21440,#12843,#12844);
#10471=AXIS2_PLACEMENT_3D('',#21443,#12846,#12847);
#10472=AXIS2_PLACEMENT_3D('',#21444,#12848,#12849);
#10473=AXIS2_PLACEMENT_3D('',#21446,#12850,#12851);
#10474=AXIS2_PLACEMENT_3D('',#21449,#12853,#12854);
#10475=AXIS2_PLACEMENT_3D('',#21450,#12855,#12856);
#10476=AXIS2_PLACEMENT_3D('',#21452,#12857,#12858);
#10477=AXIS2_PLACEMENT_3D('',#21455,#12860,#12861);
#10478=AXIS2_PLACEMENT_3D('',#21456,#12862,#12863);
#10479=AXIS2_PLACEMENT_3D('',#21458,#12864,#12865);
#10480=AXIS2_PLACEMENT_3D('',#21461,#12867,#12868);
#10481=AXIS2_PLACEMENT_3D('',#21462,#12869,#12870);
#10482=AXIS2_PLACEMENT_3D('',#21464,#12871,#12872);
#10483=AXIS2_PLACEMENT_3D('',#21467,#12874,#12875);
#10484=AXIS2_PLACEMENT_3D('',#21468,#12876,#12877);
#10485=AXIS2_PLACEMENT_3D('',#21470,#12878,#12879);
#10486=AXIS2_PLACEMENT_3D('',#21473,#12881,#12882);
#10487=AXIS2_PLACEMENT_3D('',#21474,#12883,#12884);
#10488=AXIS2_PLACEMENT_3D('',#21476,#12885,#12886);
#10489=AXIS2_PLACEMENT_3D('',#21479,#12888,#12889);
#10490=AXIS2_PLACEMENT_3D('',#21480,#12890,#12891);
#10491=AXIS2_PLACEMENT_3D('',#21482,#12892,#12893);
#10492=AXIS2_PLACEMENT_3D('',#21485,#12895,#12896);
#10493=AXIS2_PLACEMENT_3D('',#21486,#12897,#12898);
#10494=AXIS2_PLACEMENT_3D('',#21488,#12899,#12900);
#10495=AXIS2_PLACEMENT_3D('',#21491,#12902,#12903);
#10496=AXIS2_PLACEMENT_3D('',#21492,#12904,#12905);
#10497=AXIS2_PLACEMENT_3D('',#21494,#12906,#12907);
#10498=AXIS2_PLACEMENT_3D('',#21497,#12909,#12910);
#10499=AXIS2_PLACEMENT_3D('',#21498,#12911,#12912);
#10500=AXIS2_PLACEMENT_3D('',#21500,#12913,#12914);
#10501=AXIS2_PLACEMENT_3D('',#21503,#12916,#12917);
#10502=AXIS2_PLACEMENT_3D('',#21504,#12918,#12919);
#10503=AXIS2_PLACEMENT_3D('',#21506,#12920,#12921);
#10504=AXIS2_PLACEMENT_3D('',#21509,#12923,#12924);
#10505=AXIS2_PLACEMENT_3D('',#21510,#12925,#12926);
#10506=AXIS2_PLACEMENT_3D('',#21512,#12927,#12928);
#10507=AXIS2_PLACEMENT_3D('',#21515,#12930,#12931);
#10508=AXIS2_PLACEMENT_3D('',#21516,#12932,#12933);
#10509=AXIS2_PLACEMENT_3D('',#21518,#12934,#12935);
#10510=AXIS2_PLACEMENT_3D('',#21521,#12937,#12938);
#10511=AXIS2_PLACEMENT_3D('',#21522,#12939,#12940);
#10512=AXIS2_PLACEMENT_3D('',#21531,#12945,#12946);
#10513=AXIS2_PLACEMENT_3D('',#21537,#12950,#12951);
#10514=AXIS2_PLACEMENT_3D('',#21543,#12955,#12956);
#10515=AXIS2_PLACEMENT_3D('',#21546,#12959,#12960);
#10516=AXIS2_PLACEMENT_3D('',#21547,#12961,#12962);
#12769=DIRECTION('axis',(0.,0.,1.));
#12770=DIRECTION('refdir',(1.,0.,0.));
#12771=DIRECTION('center_axis',(0.,0.,1.));
#12772=DIRECTION('ref_axis',(1.,0.,0.));
#12773=DIRECTION('center_axis',(0.,0.,1.));
#12774=DIRECTION('ref_axis',(1.,0.,0.));
#12775=DIRECTION('',(0.,0.,1.));
#12776=DIRECTION('center_axis',(0.,0.,-1.));
#12777=DIRECTION('ref_axis',(1.,0.,0.));
#12778=DIRECTION('center_axis',(0.,0.,1.));
#12779=DIRECTION('ref_axis',(1.,0.,0.));
#12780=DIRECTION('center_axis',(0.,0.,1.));
#12781=DIRECTION('ref_axis',(1.,0.,0.));
#12782=DIRECTION('',(0.,0.,1.));
#12783=DIRECTION('center_axis',(0.,0.,-1.));
#12784=DIRECTION('ref_axis',(1.,0.,0.));
#12785=DIRECTION('center_axis',(0.,0.,1.));
#12786=DIRECTION('ref_axis',(1.,0.,0.));
#12787=DIRECTION('center_axis',(0.,0.,1.));
#12788=DIRECTION('ref_axis',(1.,0.,0.));
#12789=DIRECTION('',(0.,0.,1.));
#12790=DIRECTION('center_axis',(0.,0.,-1.));
#12791=DIRECTION('ref_axis',(1.,0.,0.));
#12792=DIRECTION('center_axis',(0.,0.,1.));
#12793=DIRECTION('ref_axis',(1.,0.,0.));
#12794=DIRECTION('center_axis',(0.,0.,1.));
#12795=DIRECTION('ref_axis',(1.,0.,0.));
#12796=DIRECTION('',(0.,0.,1.));
#12797=DIRECTION('center_axis',(0.,0.,-1.));
#12798=DIRECTION('ref_axis',(1.,0.,0.));
#12799=DIRECTION('center_axis',(0.,0.,1.));
#12800=DIRECTION('ref_axis',(1.,0.,0.));
#12801=DIRECTION('center_axis',(0.,0.,1.));
#12802=DIRECTION('ref_axis',(1.,0.,0.));
#12803=DIRECTION('',(0.,0.,1.));
#12804=DIRECTION('center_axis',(0.,0.,-1.));
#12805=DIRECTION('ref_axis',(1.,0.,0.));
#12806=DIRECTION('center_axis',(0.,0.,1.));
#12807=DIRECTION('ref_axis',(1.,0.,0.));
#12808=DIRECTION('center_axis',(0.,0.,1.));
#12809=DIRECTION('ref_axis',(1.,0.,0.));
#12810=DIRECTION('',(0.,0.,1.));
#12811=DIRECTION('center_axis',(0.,0.,-1.));
#12812=DIRECTION('ref_axis',(1.,0.,0.));
#12813=DIRECTION('center_axis',(0.,0.,1.));
#12814=DIRECTION('ref_axis',(1.,0.,0.));
#12815=DIRECTION('center_axis',(0.,0.,1.));
#12816=DIRECTION('ref_axis',(1.,0.,0.));
#12817=DIRECTION('',(0.,0.,1.));
#12818=DIRECTION('center_axis',(0.,0.,-1.));
#12819=DIRECTION('ref_axis',(1.,0.,0.));
#12820=DIRECTION('center_axis',(0.,0.,1.));
#12821=DIRECTION('ref_axis',(1.,0.,0.));
#12822=DIRECTION('center_axis',(0.,0.,1.));
#12823=DIRECTION('ref_axis',(1.,0.,0.));
#12824=DIRECTION('',(0.,0.,1.));
#12825=DIRECTION('center_axis',(0.,0.,-1.));
#12826=DIRECTION('ref_axis',(1.,0.,0.));
#12827=DIRECTION('center_axis',(0.,0.,1.));
#12828=DIRECTION('ref_axis',(1.,0.,0.));
#12829=DIRECTION('center_axis',(0.,0.,1.));
#12830=DIRECTION('ref_axis',(1.,0.,0.));
#12831=DIRECTION('',(0.,0.,1.));
#12832=DIRECTION('center_axis',(0.,0.,-1.));
#12833=DIRECTION('ref_axis',(1.,0.,0.));
#12834=DIRECTION('center_axis',(0.,0.,1.));
#12835=DIRECTION('ref_axis',(1.,0.,0.));
#12836=DIRECTION('center_axis',(0.,0.,1.));
#12837=DIRECTION('ref_axis',(1.,0.,0.));
#12838=DIRECTION('',(0.,0.,1.));
#12839=DIRECTION('center_axis',(0.,0.,-1.));
#12840=DIRECTION('ref_axis',(1.,0.,0.));
#12841=DIRECTION('center_axis',(0.,0.,1.));
#12842=DIRECTION('ref_axis',(1.,0.,0.));
#12843=DIRECTION('center_axis',(0.,0.,1.));
#12844=DIRECTION('ref_axis',(1.,0.,0.));
#12845=DIRECTION('',(0.,0.,1.));
#12846=DIRECTION('center_axis',(0.,0.,-1.));
#12847=DIRECTION('ref_axis',(1.,0.,0.));
#12848=DIRECTION('center_axis',(0.,0.,1.));
#12849=DIRECTION('ref_axis',(1.,0.,0.));
#12850=DIRECTION('center_axis',(0.,0.,1.));
#12851=DIRECTION('ref_axis',(1.,0.,0.));
#12852=DIRECTION('',(0.,0.,1.));
#12853=DIRECTION('center_axis',(0.,0.,-1.));
#12854=DIRECTION('ref_axis',(1.,0.,0.));
#12855=DIRECTION('center_axis',(0.,0.,1.));
#12856=DIRECTION('ref_axis',(1.,0.,0.));
#12857=DIRECTION('center_axis',(0.,0.,1.));
#12858=DIRECTION('ref_axis',(1.,0.,0.));
#12859=DIRECTION('',(0.,0.,1.));
#12860=DIRECTION('center_axis',(0.,0.,-1.));
#12861=DIRECTION('ref_axis',(1.,0.,0.));
#12862=DIRECTION('center_axis',(0.,0.,1.));
#12863=DIRECTION('ref_axis',(1.,0.,0.));
#12864=DIRECTION('center_axis',(0.,0.,1.));
#12865=DIRECTION('ref_axis',(1.,0.,0.));
#12866=DIRECTION('',(0.,0.,1.));
#12867=DIRECTION('center_axis',(0.,0.,-1.));
#12868=DIRECTION('ref_axis',(1.,0.,0.));
#12869=DIRECTION('center_axis',(0.,0.,1.));
#12870=DIRECTION('ref_axis',(1.,0.,0.));
#12871=DIRECTION('center_axis',(0.,0.,1.));
#12872=DIRECTION('ref_axis',(1.,0.,0.));
#12873=DIRECTION('',(0.,0.,1.));
#12874=DIRECTION('center_axis',(0.,0.,-1.));
#12875=DIRECTION('ref_axis',(1.,0.,0.));
#12876=DIRECTION('center_axis',(0.,0.,1.));
#12877=DIRECTION('ref_axis',(1.,0.,0.));
#12878=DIRECTION('center_axis',(0.,0.,1.));
#12879=DIRECTION('ref_axis',(1.,0.,0.));
#12880=DIRECTION('',(0.,0.,1.));
#12881=DIRECTION('center_axis',(0.,0.,-1.));
#12882=DIRECTION('ref_axis',(1.,0.,0.));
#12883=DIRECTION('center_axis',(0.,0.,1.));
#12884=DIRECTION('ref_axis',(1.,0.,0.));
#12885=DIRECTION('center_axis',(0.,0.,1.));
#12886=DIRECTION('ref_axis',(1.,0.,0.));
#12887=DIRECTION('',(0.,0.,1.));
#12888=DIRECTION('center_axis',(0.,0.,-1.));
#12889=DIRECTION('ref_axis',(1.,0.,0.));
#12890=DIRECTION('center_axis',(0.,0.,1.));
#12891=DIRECTION('ref_axis',(1.,0.,0.));
#12892=DIRECTION('center_axis',(0.,0.,1.));
#12893=DIRECTION('ref_axis',(1.,0.,0.));
#12894=DIRECTION('',(0.,0.,1.));
#12895=DIRECTION('center_axis',(0.,0.,-1.));
#12896=DIRECTION('ref_axis',(1.,0.,0.));
#12897=DIRECTION('center_axis',(0.,0.,1.));
#12898=DIRECTION('ref_axis',(1.,0.,0.));
#12899=DIRECTION('center_axis',(0.,0.,1.));
#12900=DIRECTION('ref_axis',(1.,0.,0.));
#12901=DIRECTION('',(0.,0.,1.));
#12902=DIRECTION('center_axis',(0.,0.,-1.));
#12903=DIRECTION('ref_axis',(1.,0.,0.));
#12904=DIRECTION('center_axis',(0.,0.,1.));
#12905=DIRECTION('ref_axis',(1.,0.,0.));
#12906=DIRECTION('center_axis',(0.,0.,1.));
#12907=DIRECTION('ref_axis',(1.,0.,0.));
#12908=DIRECTION('',(0.,0.,1.));
#12909=DIRECTION('center_axis',(0.,0.,-1.));
#12910=DIRECTION('ref_axis',(1.,0.,0.));
#12911=DIRECTION('center_axis',(0.,0.,1.));
#12912=DIRECTION('ref_axis',(1.,0.,0.));
#12913=DIRECTION('center_axis',(0.,0.,1.));
#12914=DIRECTION('ref_axis',(1.,0.,0.));
#12915=DIRECTION('',(0.,0.,1.));
#12916=DIRECTION('center_axis',(0.,0.,-1.));
#12917=DIRECTION('ref_axis',(1.,0.,0.));
#12918=DIRECTION('center_axis',(0.,0.,1.));
#12919=DIRECTION('ref_axis',(1.,0.,0.));
#12920=DIRECTION('center_axis',(0.,0.,1.));
#12921=DIRECTION('ref_axis',(1.,0.,0.));
#12922=DIRECTION('',(0.,0.,1.));
#12923=DIRECTION('center_axis',(0.,0.,-1.));
#12924=DIRECTION('ref_axis',(1.,0.,0.));
#12925=DIRECTION('center_axis',(0.,0.,1.));
#12926=DIRECTION('ref_axis',(1.,0.,0.));
#12927=DIRECTION('center_axis',(0.,0.,1.));
#12928=DIRECTION('ref_axis',(1.,0.,0.));
#12929=DIRECTION('',(0.,0.,1.));
#12930=DIRECTION('center_axis',(0.,0.,-1.));
#12931=DIRECTION('ref_axis',(1.,0.,0.));
#12932=DIRECTION('center_axis',(0.,0.,1.));
#12933=DIRECTION('ref_axis',(1.,0.,0.));
#12934=DIRECTION('center_axis',(0.,0.,1.));
#12935=DIRECTION('ref_axis',(1.,0.,0.));
#12936=DIRECTION('',(0.,0.,1.));
#12937=DIRECTION('center_axis',(0.,0.,-1.));
#12938=DIRECTION('ref_axis',(1.,0.,0.));
#12939=DIRECTION('center_axis',(0.,1.,0.));
#12940=DIRECTION('ref_axis',(-1.,0.,0.));
#12941=DIRECTION('',(-1.,0.,0.));
#12942=DIRECTION('',(0.,0.,1.));
#12943=DIRECTION('',(-1.,0.,0.));
#12944=DIRECTION('',(0.,0.,1.));
#12945=DIRECTION('center_axis',(1.,0.,0.));
#12946=DIRECTION('ref_axis',(0.,1.,0.));
#12947=DIRECTION('',(0.,1.,0.));
#12948=DIRECTION('',(0.,1.,0.));
#12949=DIRECTION('',(0.,0.,1.));
#12950=DIRECTION('center_axis',(0.,-1.,0.));
#12951=DIRECTION('ref_axis',(1.,0.,0.));
#12952=DIRECTION('',(1.,0.,0.));
#12953=DIRECTION('',(1.,0.,0.));
#12954=DIRECTION('',(0.,0.,1.));
#12955=DIRECTION('center_axis',(-1.,0.,0.));
#12956=DIRECTION('ref_axis',(0.,-1.,0.));
#12957=DIRECTION('',(0.,-1.,0.));
#12958=DIRECTION('',(0.,-1.,0.));
#12959=DIRECTION('center_axis',(0.,0.,1.));
#12960=DIRECTION('ref_axis',(1.,0.,0.));
#12961=DIRECTION('center_axis',(0.,0.,1.));
#12962=DIRECTION('ref_axis',(1.,0.,0.));
#21377=CARTESIAN_POINT('',(0.,0.,0.));
#21378=CARTESIAN_POINT('Origin',(0.,-1.,15.));
#21379=CARTESIAN_POINT('',(-0.225,-1.,15.1));
#21380=CARTESIAN_POINT('Origin',(0.,-1.,15.1));
#21381=CARTESIAN_POINT('',(-0.225,-1.,16.3));
#21382=CARTESIAN_POINT('',(-0.225,-1.,15.));
#21383=CARTESIAN_POINT('Origin',(0.,-1.,16.3));
#21384=CARTESIAN_POINT('Origin',(1.,0.,15.));
#21385=CARTESIAN_POINT('',(0.775,-2.75545529808155E-17,15.1));
#21386=CARTESIAN_POINT('Origin',(1.,0.,15.1));
#21387=CARTESIAN_POINT('',(0.775,2.75545529808155E-17,16.3));
#21388=CARTESIAN_POINT('',(0.775,-2.75545529808155E-17,15.));
#21389=CARTESIAN_POINT('Origin',(1.,0.,16.3));
#21390=CARTESIAN_POINT('Origin',(-1.,0.,15.));
#21391=CARTESIAN_POINT('',(-1.225,-2.75545529808154E-17,15.1));
#21392=CARTESIAN_POINT('Origin',(-1.,0.,15.1));
#21393=CARTESIAN_POINT('',(-1.225,2.75545529808154E-17,16.3));
#21394=CARTESIAN_POINT('',(-1.225,-2.75545529808154E-17,15.));
#21395=CARTESIAN_POINT('Origin',(-1.,0.,16.3));
#21396=CARTESIAN_POINT('Origin',(0.,1.,15.));
#21397=CARTESIAN_POINT('',(-0.225,1.,15.1));
#21398=CARTESIAN_POINT('Origin',(0.,1.,15.1));
#21399=CARTESIAN_POINT('',(-0.225,1.,16.3));
#21400=CARTESIAN_POINT('',(-0.225,1.,15.));
#21401=CARTESIAN_POINT('Origin',(0.,1.,16.3));
#21402=CARTESIAN_POINT('Origin',(4.86862915010152,2.86862915010152,15.));
#21403=CARTESIAN_POINT('',(4.64362915010152,2.86862915010152,15.1));
#21404=CARTESIAN_POINT('Origin',(4.86862915010152,2.86862915010152,15.1));
#21405=CARTESIAN_POINT('',(4.64362915010152,2.86862915010152,16.3));
#21406=CARTESIAN_POINT('',(4.64362915010152,2.86862915010152,15.));
#21407=CARTESIAN_POINT('Origin',(4.86862915010152,2.86862915010152,16.3));
#21408=CARTESIAN_POINT('Origin',(4.86862915010152,5.13137084989848,15.));
#21409=CARTESIAN_POINT('',(4.64362915010152,5.13137084989848,15.1));
#21410=CARTESIAN_POINT('Origin',(4.86862915010152,5.13137084989848,15.1));
#21411=CARTESIAN_POINT('',(4.64362915010152,5.13137084989848,16.3));
#21412=CARTESIAN_POINT('',(4.64362915010152,5.13137084989848,15.));
#21413=CARTESIAN_POINT('Origin',(4.86862915010152,5.13137084989848,16.3));
#21414=CARTESIAN_POINT('Origin',(7.13137084989848,5.13137084989848,15.));
#21415=CARTESIAN_POINT('',(6.90637084989848,5.13137084989848,15.1));
#21416=CARTESIAN_POINT('Origin',(7.13137084989848,5.13137084989848,15.1));
#21417=CARTESIAN_POINT('',(6.90637084989848,5.13137084989848,16.3));
#21418=CARTESIAN_POINT('',(6.90637084989848,5.13137084989848,15.));
#21419=CARTESIAN_POINT('Origin',(7.13137084989848,5.13137084989848,16.3));
#21420=CARTESIAN_POINT('Origin',(7.13137084989848,2.86862915010152,15.));
#21421=CARTESIAN_POINT('',(6.90637084989848,2.86862915010152,15.1));
#21422=CARTESIAN_POINT('Origin',(7.13137084989848,2.86862915010152,15.1));
#21423=CARTESIAN_POINT('',(6.90637084989848,2.86862915010152,16.3));
#21424=CARTESIAN_POINT('',(6.90637084989848,2.86862915010152,15.));
#21425=CARTESIAN_POINT('Origin',(7.13137084989848,2.86862915010152,16.3));
#21426=CARTESIAN_POINT('Origin',(4.86862915010152,-5.13137084989848,15.));
#21427=CARTESIAN_POINT('',(4.64362915010152,-5.13137084989848,15.1));
#21428=CARTESIAN_POINT('Origin',(4.86862915010152,-5.13137084989848,15.1));
#21429=CARTESIAN_POINT('',(4.64362915010152,-5.13137084989848,16.3));
#21430=CARTESIAN_POINT('',(4.64362915010152,-5.13137084989848,15.));
#21431=CARTESIAN_POINT('Origin',(4.86862915010152,-5.13137084989848,16.3));
#21432=CARTESIAN_POINT('Origin',(4.86862915010152,-2.86862915010152,15.));
#21433=CARTESIAN_POINT('',(4.64362915010152,-2.86862915010152,15.1));
#21434=CARTESIAN_POINT('Origin',(4.86862915010152,-2.86862915010152,15.1));
#21435=CARTESIAN_POINT('',(4.64362915010152,-2.86862915010152,16.3));
#21436=CARTESIAN_POINT('',(4.64362915010152,-2.86862915010152,15.));
#21437=CARTESIAN_POINT('Origin',(4.86862915010152,-2.86862915010152,16.3));
#21438=CARTESIAN_POINT('Origin',(7.13137084989848,-2.86862915010152,15.));
#21439=CARTESIAN_POINT('',(6.90637084989848,-2.86862915010152,15.1));
#21440=CARTESIAN_POINT('Origin',(7.13137084989848,-2.86862915010152,15.1));
#21441=CARTESIAN_POINT('',(6.90637084989848,-2.86862915010152,16.3));
#21442=CARTESIAN_POINT('',(6.90637084989848,-2.86862915010152,15.));
#21443=CARTESIAN_POINT('Origin',(7.13137084989848,-2.86862915010152,16.3));
#21444=CARTESIAN_POINT('Origin',(7.13137084989848,-5.13137084989848,15.));
#21445=CARTESIAN_POINT('',(6.90637084989848,-5.13137084989848,15.1));
#21446=CARTESIAN_POINT('Origin',(7.13137084989848,-5.13137084989848,15.1));
#21447=CARTESIAN_POINT('',(6.90637084989848,-5.13137084989848,16.3));
#21448=CARTESIAN_POINT('',(6.90637084989848,-5.13137084989848,15.));
#21449=CARTESIAN_POINT('Origin',(7.13137084989848,-5.13137084989848,16.3));
#21450=CARTESIAN_POINT('Origin',(-7.13137084989848,2.86862915010152,15.));
#21451=CARTESIAN_POINT('',(-7.35637084989848,2.86862915010152,15.1));
#21452=CARTESIAN_POINT('Origin',(-7.13137084989848,2.86862915010152,15.1));
#21453=CARTESIAN_POINT('',(-7.35637084989848,2.86862915010152,16.3));
#21454=CARTESIAN_POINT('',(-7.35637084989848,2.86862915010152,15.));
#21455=CARTESIAN_POINT('Origin',(-7.13137084989848,2.86862915010152,16.3));
#21456=CARTESIAN_POINT('Origin',(-7.13137084989848,5.13137084989848,15.));
#21457=CARTESIAN_POINT('',(-7.35637084989848,5.13137084989848,15.1));
#21458=CARTESIAN_POINT('Origin',(-7.13137084989848,5.13137084989848,15.1));
#21459=CARTESIAN_POINT('',(-7.35637084989848,5.13137084989848,16.3));
#21460=CARTESIAN_POINT('',(-7.35637084989848,5.13137084989848,15.));
#21461=CARTESIAN_POINT('Origin',(-7.13137084989848,5.13137084989848,16.3));
#21462=CARTESIAN_POINT('Origin',(-4.86862915010152,5.13137084989848,15.));
#21463=CARTESIAN_POINT('',(-5.09362915010152,5.13137084989848,15.1));
#21464=CARTESIAN_POINT('Origin',(-4.86862915010152,5.13137084989848,15.1));
#21465=CARTESIAN_POINT('',(-5.09362915010152,5.13137084989848,16.3));
#21466=CARTESIAN_POINT('',(-5.09362915010152,5.13137084989848,15.));
#21467=CARTESIAN_POINT('Origin',(-4.86862915010152,5.13137084989848,16.3));
#21468=CARTESIAN_POINT('Origin',(-4.86862915010152,2.86862915010152,15.));
#21469=CARTESIAN_POINT('',(-5.09362915010152,2.86862915010152,15.1));
#21470=CARTESIAN_POINT('Origin',(-4.86862915010152,2.86862915010152,15.1));
#21471=CARTESIAN_POINT('',(-5.09362915010152,2.86862915010152,16.3));
#21472=CARTESIAN_POINT('',(-5.09362915010152,2.86862915010152,15.));
#21473=CARTESIAN_POINT('Origin',(-4.86862915010152,2.86862915010152,16.3));
#21474=CARTESIAN_POINT('Origin',(-7.13137084989848,-5.13137084989848,15.));
#21475=CARTESIAN_POINT('',(-7.35637084989848,-5.13137084989848,15.1));
#21476=CARTESIAN_POINT('Origin',(-7.13137084989848,-5.13137084989848,15.1));
#21477=CARTESIAN_POINT('',(-7.35637084989848,-5.13137084989848,16.3));
#21478=CARTESIAN_POINT('',(-7.35637084989848,-5.13137084989848,15.));
#21479=CARTESIAN_POINT('Origin',(-7.13137084989848,-5.13137084989848,16.3));
#21480=CARTESIAN_POINT('Origin',(-7.13137084989848,-2.86862915010152,15.));
#21481=CARTESIAN_POINT('',(-7.35637084989848,-2.86862915010152,15.1));
#21482=CARTESIAN_POINT('Origin',(-7.13137084989848,-2.86862915010152,15.1));
#21483=CARTESIAN_POINT('',(-7.35637084989848,-2.86862915010152,16.3));
#21484=CARTESIAN_POINT('',(-7.35637084989848,-2.86862915010152,15.));
#21485=CARTESIAN_POINT('Origin',(-7.13137084989848,-2.86862915010152,16.3));
#21486=CARTESIAN_POINT('Origin',(-4.86862915010152,-2.86862915010152,15.));
#21487=CARTESIAN_POINT('',(-5.09362915010152,-2.86862915010152,15.1));
#21488=CARTESIAN_POINT('Origin',(-4.86862915010152,-2.86862915010152,15.1));
#21489=CARTESIAN_POINT('',(-5.09362915010152,-2.86862915010152,16.3));
#21490=CARTESIAN_POINT('',(-5.09362915010152,-2.86862915010152,15.));
#21491=CARTESIAN_POINT('Origin',(-4.86862915010152,-2.86862915010152,16.3));
#21492=CARTESIAN_POINT('Origin',(-4.86862915010152,-5.13137084989848,15.));
#21493=CARTESIAN_POINT('',(-5.09362915010152,-5.13137084989848,15.1));
#21494=CARTESIAN_POINT('Origin',(-4.86862915010152,-5.13137084989848,15.1));
#21495=CARTESIAN_POINT('',(-5.09362915010152,-5.13137084989848,16.3));
#21496=CARTESIAN_POINT('',(-5.09362915010152,-5.13137084989848,15.));
#21497=CARTESIAN_POINT('Origin',(-4.86862915010152,-5.13137084989848,16.3));
#21498=CARTESIAN_POINT('Origin',(6.,-4.,15.));
#21499=CARTESIAN_POINT('',(5.375,-4.,15.1));
#21500=CARTESIAN_POINT('Origin',(6.,-4.,15.1));
#21501=CARTESIAN_POINT('',(5.375,-4.,16.3));
#21502=CARTESIAN_POINT('',(5.375,-4.,15.));
#21503=CARTESIAN_POINT('Origin',(6.,-4.,16.3));
#21504=CARTESIAN_POINT('Origin',(-6.,4.,15.));
#21505=CARTESIAN_POINT('',(-6.625,4.,15.1));
#21506=CARTESIAN_POINT('Origin',(-6.,4.,15.1));
#21507=CARTESIAN_POINT('',(-6.625,4.,16.3));
#21508=CARTESIAN_POINT('',(-6.625,4.,15.));
#21509=CARTESIAN_POINT('Origin',(-6.,4.,16.3));
#21510=CARTESIAN_POINT('Origin',(-6.,-4.,15.));
#21511=CARTESIAN_POINT('',(-6.625,-4.,15.1));
#21512=CARTESIAN_POINT('Origin',(-6.,-4.,15.1));
#21513=CARTESIAN_POINT('',(-6.625,-4.,16.3));
#21514=CARTESIAN_POINT('',(-6.625,-4.,15.));
#21515=CARTESIAN_POINT('Origin',(-6.,-4.,16.3));
#21516=CARTESIAN_POINT('Origin',(6.,4.,15.));
#21517=CARTESIAN_POINT('',(5.375,4.,15.1));
#21518=CARTESIAN_POINT('Origin',(6.,4.,15.1));
#21519=CARTESIAN_POINT('',(5.375,4.,16.3));
#21520=CARTESIAN_POINT('',(5.375,4.,15.));
#21521=CARTESIAN_POINT('Origin',(6.,4.,16.3));
#21522=CARTESIAN_POINT('Origin',(8.5,6.5,15.1));
#21523=CARTESIAN_POINT('',(8.5,6.5,15.1));
#21524=CARTESIAN_POINT('',(-8.5,6.5,15.1));
#21525=CARTESIAN_POINT('',(8.5,6.5,15.1));
#21526=CARTESIAN_POINT('',(-8.5,6.5,16.3));
#21527=CARTESIAN_POINT('',(-8.5,6.5,15.1));
#21528=CARTESIAN_POINT('',(8.5,6.5,16.3));
#21529=CARTESIAN_POINT('',(8.5,6.5,16.3));
#21530=CARTESIAN_POINT('',(8.5,6.5,15.1));
#21531=CARTESIAN_POINT('Origin',(8.5,-6.5,15.1));
#21532=CARTESIAN_POINT('',(8.5,-6.5,15.1));
#21533=CARTESIAN_POINT('',(8.5,-6.5,15.1));
#21534=CARTESIAN_POINT('',(8.5,-6.5,16.3));
#21535=CARTESIAN_POINT('',(8.5,-6.5,16.3));
#21536=CARTESIAN_POINT('',(8.5,-6.5,15.1));
#21537=CARTESIAN_POINT('Origin',(-8.5,-6.5,15.1));
#21538=CARTESIAN_POINT('',(-8.5,-6.5,15.1));
#21539=CARTESIAN_POINT('',(-8.5,-6.5,15.1));
#21540=CARTESIAN_POINT('',(-8.5,-6.5,16.3));
#21541=CARTESIAN_POINT('',(-8.5,-6.5,16.3));
#21542=CARTESIAN_POINT('',(-8.5,-6.5,15.1));
#21543=CARTESIAN_POINT('Origin',(-8.5,6.5,15.1));
#21544=CARTESIAN_POINT('',(-8.5,6.5,15.1));
#21545=CARTESIAN_POINT('',(-8.5,6.5,16.3));
#21546=CARTESIAN_POINT('Origin',(0.,0.,16.3));
#21547=CARTESIAN_POINT('Origin',(0.,0.,15.1));
#22333=UNCERTAINTY_MEASURE_WITH_UNIT(LENGTH_MEASURE(0.001),#22395,
'DISTANCE_ACCURACY_VALUE',
'Maximum model space distance between geometric entities at asserted c
onnectivities');
#22343=UNCERTAINTY_MEASURE_WITH_UNIT(LENGTH_MEASURE(0.001),#22395,
'DISTANCE_ACCURACY_VALUE',
'Maximum model space distance between geometric entities at asserted c
onnectivities');
#22384=(
GEOMETRIC_REPRESENTATION_CONTEXT(3)
GLOBAL_UNCERTAINTY_ASSIGNED_CONTEXT((#22333))
GLOBAL_UNIT_ASSIGNED_CONTEXT((#22395,#22397,#22398))
REPRESENTATION_CONTEXT('','3D')
);
#22394=(
GEOMETRIC_REPRESENTATION_CONTEXT(3)
GLOBAL_UNCERTAINTY_ASSIGNED_CONTEXT((#22343))
GLOBAL_UNIT_ASSIGNED_CONTEXT((#22395,#22397,#22398))
REPRESENTATION_CONTEXT('','3D')
);
#22395=(
LENGTH_UNIT()
NAMED_UNIT(*)
SI_UNIT(.CENTI.,.METRE.)
);
#22397=(
NAMED_UNIT(*)
PLANE_ANGLE_UNIT()
SI_UNIT($,.RADIAN.)
);
#22398=(
NAMED_UNIT(*)
SI_UNIT($,.STERADIAN.)
SOLID_ANGLE_UNIT()
);
#22439=SHAPE_DEFINITION_REPRESENTATION(#22489,#22678);
#22489=PRODUCT_DEFINITION_SHAPE('',$,#22729);
#22678=SHAPE_REPRESENTATION('',(#10438),#22384);
#22688=PRODUCT_DEFINITION_CONTEXT('part definition',#22840,'design');
#22729=PRODUCT_DEFINITION('Table','Table',#22779,#22688);
#22779=PRODUCT_DEFINITION_FORMATION('',$,#22882);
#22840=APPLICATION_CONTEXT(
'Core Data for Automotive Mechanical Design Process');
#22841=PRODUCT_CONTEXT('part definition',#22840,'mechanical');
#22882=PRODUCT('Table','Table','Table',(#22841));
#22969=COLOUR_RGB('Off White',0.89,0.88,0.83);
#22970=FILL_AREA_STYLE_COLOUR('',#22969);
#22971=FILL_AREA_STYLE('',(#22970));
#22972=SURFACE_STYLE_FILL_AREA(#22971);
#22973=SURFACE_SIDE_STYLE('',(#22972));
#22974=SURFACE_STYLE_USAGE(.BOTH.,#22973);
#22975=PRESENTATION_STYLE_ASSIGNMENT((#22974));
ENDSEC;
END-ISO-10303-21;
